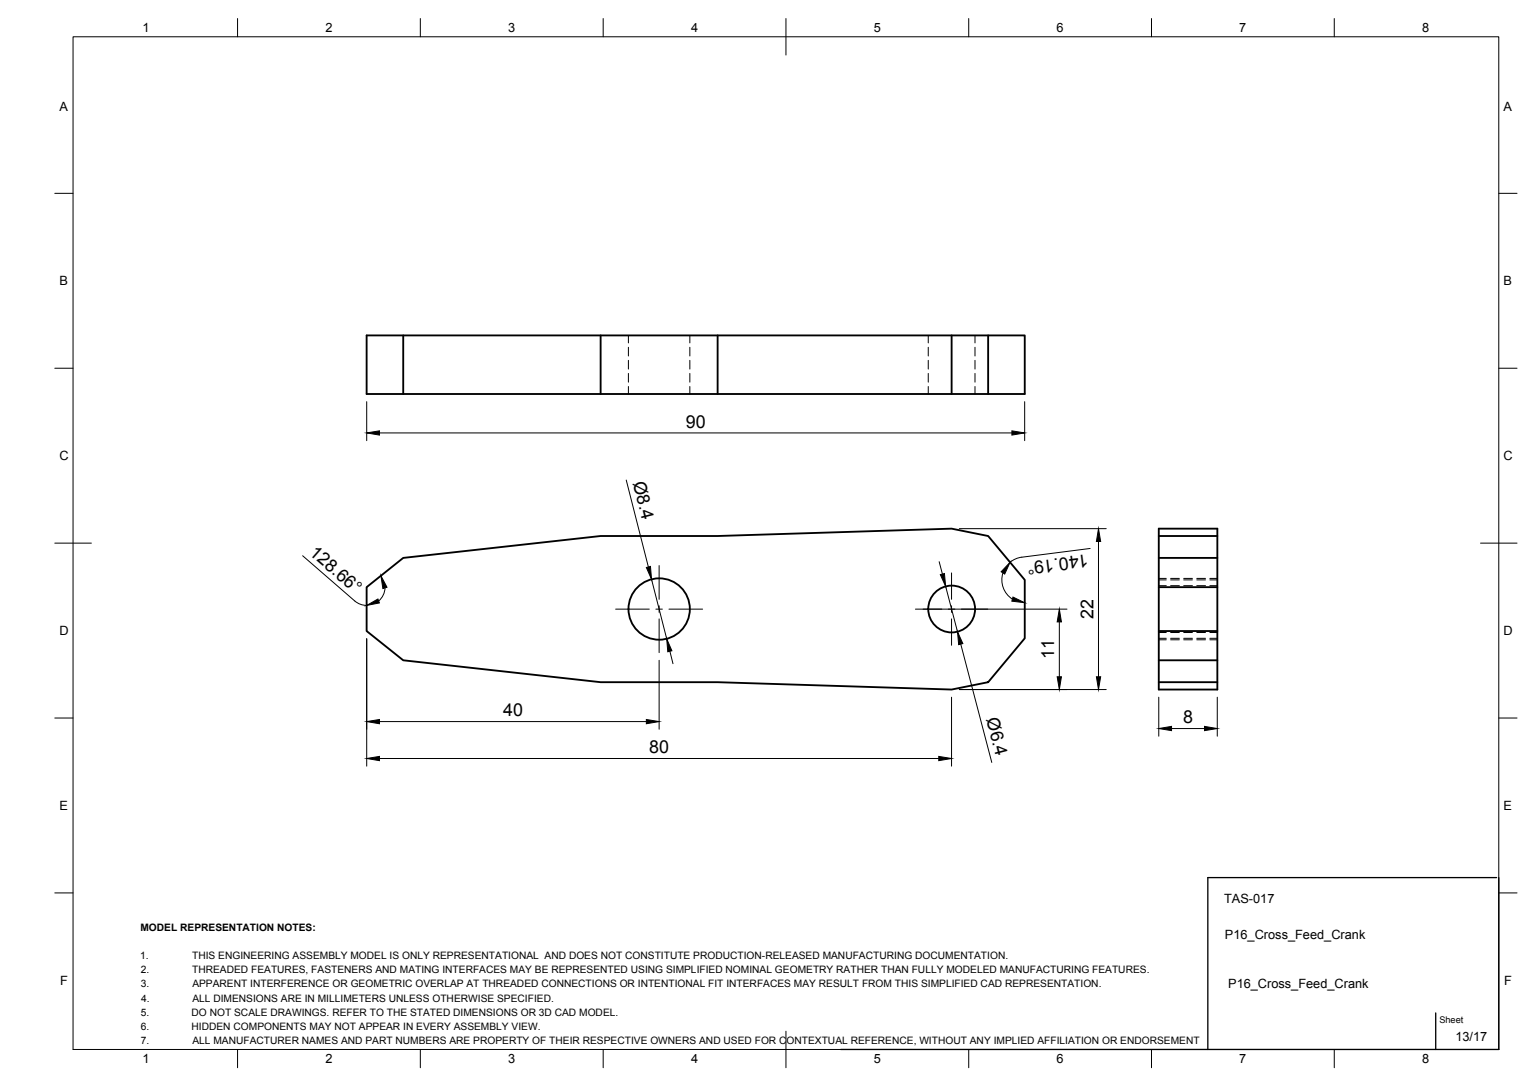
ISO-10303-21;
HEADER;
/* Generated by software containing ST-Developer
 * from STEP Tools, Inc. (www.steptools.com) 
 */

FILE_DESCRIPTION(
/* description */ ('STEP AP203'),
/* implementation_level */ '2;1');

FILE_NAME(
/* name */ 'P16_Cross_Feed_Crank.step',
/* time_stamp */ '2026-11-15T15:04:01-08:00',
/* author */ (''),
/* organization */ (''),
/* preprocessor_version */ 'ST-DEVELOPER v20.2',
/* originating_system */ 'Autodesk Translation Framework v15.17.0.0',
/* authorisation */ '');

FILE_SCHEMA (('AUTOMOTIVE_DESIGN { 1 0 10303 214 3 1 1 }'));
ENDSEC;

DATA;
#10=MECHANICAL_DESIGN_GEOMETRIC_PRESENTATION_REPRESENTATION('',(#299),#16598);
#221=SHAPE_REPRESENTATION_RELATIONSHIP('SRR','None',#16715,#245);
#245=ADVANCED_BREP_SHAPE_REPRESENTATION('',(#269),#16591);
#269=MANIFOLD_SOLID_BREP('Body1',#9804);
#299=STYLED_ITEM('',(#16830),#269);
#415=FACE_BOUND('',#2053,.T.);
#416=FACE_BOUND('',#2054,.T.);
#417=FACE_BOUND('',#2056,.T.);
#418=FACE_BOUND('',#2057,.T.);
#853=PLANE('',#10785);
#854=PLANE('',#10786);
#855=PLANE('',#10787);
#856=PLANE('',#10788);
#857=PLANE('',#10789);
#858=PLANE('',#10790);
#859=PLANE('',#10791);
#860=PLANE('',#10792);
#861=PLANE('',#10793);
#862=PLANE('',#10794);
#863=PLANE('',#10795);
#864=PLANE('',#10796);
#865=PLANE('',#10797);
#866=PLANE('',#10798);
#867=PLANE('',#10799);
#868=PLANE('',#10800);
#1390=FACE_OUTER_BOUND('',#2050,.T.);
#1391=FACE_OUTER_BOUND('',#2051,.T.);
#1392=FACE_OUTER_BOUND('',#2052,.T.);
#1393=FACE_OUTER_BOUND('',#2055,.T.);
#1394=FACE_OUTER_BOUND('',#2058,.T.);
#1395=FACE_OUTER_BOUND('',#2059,.T.);
#1396=FACE_OUTER_BOUND('',#2060,.T.);
#1397=FACE_OUTER_BOUND('',#2061,.T.);
#1398=FACE_OUTER_BOUND('',#2062,.T.);
#1399=FACE_OUTER_BOUND('',#2063,.T.);
#1400=FACE_OUTER_BOUND('',#2064,.T.);
#1401=FACE_OUTER_BOUND('',#2065,.T.);
#1402=FACE_OUTER_BOUND('',#2066,.T.);
#1403=FACE_OUTER_BOUND('',#2067,.T.);
#1404=FACE_OUTER_BOUND('',#2068,.T.);
#1405=FACE_OUTER_BOUND('',#2069,.T.);
#1406=FACE_OUTER_BOUND('',#2070,.T.);
#1407=FACE_OUTER_BOUND('',#2071,.T.);
#2050=EDGE_LOOP('',(#8859,#8860,#8861,#8862));
#2051=EDGE_LOOP('',(#8863,#8864,#8865,#8866));
#2052=EDGE_LOOP('',(#8867,#8868,#8869,#8870,#8871,#8872,#8873,#8874,#8875,
#8876,#8877,#8878,#8879,#8880));
#2053=EDGE_LOOP('',(#8881));
#2054=EDGE_LOOP('',(#8882));
#2055=EDGE_LOOP('',(#8883,#8884,#8885,#8886,#8887,#8888,#8889,#8890,#8891,
#8892,#8893,#8894,#8895,#8896));
#2056=EDGE_LOOP('',(#8897));
#2057=EDGE_LOOP('',(#8898));
#2058=EDGE_LOOP('',(#8899,#8900,#8901,#8902));
#2059=EDGE_LOOP('',(#8903,#8904,#8905,#8906));
#2060=EDGE_LOOP('',(#8907,#8908,#8909,#8910));
#2061=EDGE_LOOP('',(#8911,#8912,#8913,#8914));
#2062=EDGE_LOOP('',(#8915,#8916,#8917,#8918));
#2063=EDGE_LOOP('',(#8919,#8920,#8921,#8922));
#2064=EDGE_LOOP('',(#8923,#8924,#8925,#8926));
#2065=EDGE_LOOP('',(#8927,#8928,#8929,#8930));
#2066=EDGE_LOOP('',(#8931,#8932,#8933,#8934));
#2067=EDGE_LOOP('',(#8935,#8936,#8937,#8938));
#2068=EDGE_LOOP('',(#8939,#8940,#8941,#8942));
#2069=EDGE_LOOP('',(#8943,#8944,#8945,#8946));
#2070=EDGE_LOOP('',(#8947,#8948,#8949,#8950));
#2071=EDGE_LOOP('',(#8951,#8952,#8953,#8954));
#3056=LINE('',#16171,#4104);
#3057=LINE('',#16177,#4105);
#3058=LINE('',#16182,#4106);
#3059=LINE('',#16184,#4107);
#3060=LINE('',#16186,#4108);
#3061=LINE('',#16188,#4109);
#3062=LINE('',#16190,#4110);
#3063=LINE('',#16192,#4111);
#3064=LINE('',#16194,#4112);
#3065=LINE('',#16196,#4113);
#3066=LINE('',#16198,#4114);
#3067=LINE('',#16200,#4115);
#3068=LINE('',#16202,#4116);
#3069=LINE('',#16204,#4117);
#3070=LINE('',#16206,#4118);
#3071=LINE('',#16207,#4119);
#3072=LINE('',#16211,#4120);
#3073=LINE('',#16213,#4121);
#3074=LINE('',#16215,#4122);
#3075=LINE('',#16217,#4123);
#3076=LINE('',#16219,#4124);
#3077=LINE('',#16221,#4125);
#3078=LINE('',#16223,#4126);
#3079=LINE('',#16225,#4127);
#3080=LINE('',#16227,#4128);
#3081=LINE('',#16229,#4129);
#3082=LINE('',#16231,#4130);
#3083=LINE('',#16233,#4131);
#3084=LINE('',#16235,#4132);
#3085=LINE('',#16236,#4133);
#3086=LINE('',#16238,#4134);
#3087=LINE('',#16239,#4135);
#3088=LINE('',#16241,#4136);
#3089=LINE('',#16243,#4137);
#3090=LINE('',#16245,#4138);
#3091=LINE('',#16247,#4139);
#3092=LINE('',#16249,#4140);
#3093=LINE('',#16251,#4141);
#3094=LINE('',#16253,#4142);
#3095=LINE('',#16255,#4143);
#3096=LINE('',#16257,#4144);
#3097=LINE('',#16259,#4145);
#3098=LINE('',#16261,#4146);
#3099=LINE('',#16263,#4147);
#4104=VECTOR('',#13258,3.2);
#4105=VECTOR('',#13265,4.2);
#4106=VECTOR('',#13270,1000.);
#4107=VECTOR('',#13271,1000.);
#4108=VECTOR('',#13272,1000.);
#4109=VECTOR('',#13273,1000.);
#4110=VECTOR('',#13274,1000.);
#4111=VECTOR('',#13275,1000.);
#4112=VECTOR('',#13276,1000.);
#4113=VECTOR('',#13277,1000.);
#4114=VECTOR('',#13278,1000.);
#4115=VECTOR('',#13279,1000.);
#4116=VECTOR('',#13280,1000.);
#4117=VECTOR('',#13281,1000.);
#4118=VECTOR('',#13282,1000.);
#4119=VECTOR('',#13283,1000.);
#4120=VECTOR('',#13286,1000.);
#4121=VECTOR('',#13287,1000.);
#4122=VECTOR('',#13288,1000.);
#4123=VECTOR('',#13289,1000.);
#4124=VECTOR('',#13290,1000.);
#4125=VECTOR('',#13291,1000.);
#4126=VECTOR('',#13292,1000.);
#4127=VECTOR('',#13293,1000.);
#4128=VECTOR('',#13294,1000.);
#4129=VECTOR('',#13295,1000.);
#4130=VECTOR('',#13296,1000.);
#4131=VECTOR('',#13297,1000.);
#4132=VECTOR('',#13298,1000.);
#4133=VECTOR('',#13299,1000.);
#4134=VECTOR('',#13302,1000.);
#4135=VECTOR('',#13303,1000.);
#4136=VECTOR('',#13306,1000.);
#4137=VECTOR('',#13309,1000.);
#4138=VECTOR('',#13312,1000.);
#4139=VECTOR('',#13315,1000.);
#4140=VECTOR('',#13318,1000.);
#4141=VECTOR('',#13321,1000.);
#4142=VECTOR('',#13324,1000.);
#4143=VECTOR('',#13327,1000.);
#4144=VECTOR('',#13330,1000.);
#4145=VECTOR('',#13333,1000.);
#4146=VECTOR('',#13336,1000.);
#4147=VECTOR('',#13339,1000.);
#4428=CIRCLE('',#10780,3.2);
#4429=CIRCLE('',#10781,3.2);
#4430=CIRCLE('',#10783,4.2);
#4431=CIRCLE('',#10784,4.2);
#5208=VERTEX_POINT('',#16168);
#5209=VERTEX_POINT('',#16170);
#5210=VERTEX_POINT('',#16174);
#5211=VERTEX_POINT('',#16176);
#5212=VERTEX_POINT('',#16180);
#5213=VERTEX_POINT('',#16181);
#5214=VERTEX_POINT('',#16183);
#5215=VERTEX_POINT('',#16185);
#5216=VERTEX_POINT('',#16187);
#5217=VERTEX_POINT('',#16189);
#5218=VERTEX_POINT('',#16191);
#5219=VERTEX_POINT('',#16193);
#5220=VERTEX_POINT('',#16195);
#5221=VERTEX_POINT('',#16197);
#5222=VERTEX_POINT('',#16199);
#5223=VERTEX_POINT('',#16201);
#5224=VERTEX_POINT('',#16203);
#5225=VERTEX_POINT('',#16205);
#5226=VERTEX_POINT('',#16209);
#5227=VERTEX_POINT('',#16210);
#5228=VERTEX_POINT('',#16212);
#5229=VERTEX_POINT('',#16214);
#5230=VERTEX_POINT('',#16216);
#5231=VERTEX_POINT('',#16218);
#5232=VERTEX_POINT('',#16220);
#5233=VERTEX_POINT('',#16222);
#5234=VERTEX_POINT('',#16224);
#5235=VERTEX_POINT('',#16226);
#5236=VERTEX_POINT('',#16228);
#5237=VERTEX_POINT('',#16230);
#5238=VERTEX_POINT('',#16232);
#5239=VERTEX_POINT('',#16234);
#6442=EDGE_CURVE('',#5208,#5208,#4428,.T.);
#6443=EDGE_CURVE('',#5208,#5209,#3056,.T.);
#6444=EDGE_CURVE('',#5209,#5209,#4429,.T.);
#6445=EDGE_CURVE('',#5210,#5210,#4430,.T.);
#6446=EDGE_CURVE('',#5210,#5211,#3057,.T.);
#6447=EDGE_CURVE('',#5211,#5211,#4431,.T.);
#6448=EDGE_CURVE('',#5212,#5213,#3058,.T.);
#6449=EDGE_CURVE('',#5213,#5214,#3059,.T.);
#6450=EDGE_CURVE('',#5214,#5215,#3060,.T.);
#6451=EDGE_CURVE('',#5215,#5216,#3061,.T.);
#6452=EDGE_CURVE('',#5216,#5217,#3062,.T.);
#6453=EDGE_CURVE('',#5217,#5218,#3063,.T.);
#6454=EDGE_CURVE('',#5218,#5219,#3064,.T.);
#6455=EDGE_CURVE('',#5219,#5220,#3065,.T.);
#6456=EDGE_CURVE('',#5220,#5221,#3066,.T.);
#6457=EDGE_CURVE('',#5221,#5222,#3067,.T.);
#6458=EDGE_CURVE('',#5222,#5223,#3068,.T.);
#6459=EDGE_CURVE('',#5223,#5224,#3069,.T.);
#6460=EDGE_CURVE('',#5224,#5225,#3070,.T.);
#6461=EDGE_CURVE('',#5225,#5212,#3071,.T.);
#6462=EDGE_CURVE('',#5226,#5227,#3072,.T.);
#6463=EDGE_CURVE('',#5228,#5226,#3073,.T.);
#6464=EDGE_CURVE('',#5229,#5228,#3074,.T.);
#6465=EDGE_CURVE('',#5230,#5229,#3075,.T.);
#6466=EDGE_CURVE('',#5231,#5230,#3076,.T.);
#6467=EDGE_CURVE('',#5232,#5231,#3077,.T.);
#6468=EDGE_CURVE('',#5233,#5232,#3078,.T.);
#6469=EDGE_CURVE('',#5234,#5233,#3079,.T.);
#6470=EDGE_CURVE('',#5235,#5234,#3080,.T.);
#6471=EDGE_CURVE('',#5236,#5235,#3081,.T.);
#6472=EDGE_CURVE('',#5237,#5236,#3082,.T.);
#6473=EDGE_CURVE('',#5238,#5237,#3083,.T.);
#6474=EDGE_CURVE('',#5239,#5238,#3084,.T.);
#6475=EDGE_CURVE('',#5227,#5239,#3085,.T.);
#6476=EDGE_CURVE('',#5213,#5227,#3086,.T.);
#6477=EDGE_CURVE('',#5212,#5226,#3087,.T.);
#6478=EDGE_CURVE('',#5214,#5239,#3088,.T.);
#6479=EDGE_CURVE('',#5215,#5238,#3089,.T.);
#6480=EDGE_CURVE('',#5216,#5237,#3090,.T.);
#6481=EDGE_CURVE('',#5217,#5236,#3091,.T.);
#6482=EDGE_CURVE('',#5218,#5235,#3092,.T.);
#6483=EDGE_CURVE('',#5219,#5234,#3093,.T.);
#6484=EDGE_CURVE('',#5220,#5233,#3094,.T.);
#6485=EDGE_CURVE('',#5221,#5232,#3095,.T.);
#6486=EDGE_CURVE('',#5222,#5231,#3096,.T.);
#6487=EDGE_CURVE('',#5223,#5230,#3097,.T.);
#6488=EDGE_CURVE('',#5224,#5229,#3098,.T.);
#6489=EDGE_CURVE('',#5225,#5228,#3099,.T.);
#8859=ORIENTED_EDGE('',*,*,#6442,.T.);
#8860=ORIENTED_EDGE('',*,*,#6443,.T.);
#8861=ORIENTED_EDGE('',*,*,#6444,.F.);
#8862=ORIENTED_EDGE('',*,*,#6443,.F.);
#8863=ORIENTED_EDGE('',*,*,#6445,.T.);
#8864=ORIENTED_EDGE('',*,*,#6446,.T.);
#8865=ORIENTED_EDGE('',*,*,#6447,.F.);
#8866=ORIENTED_EDGE('',*,*,#6446,.F.);
#8867=ORIENTED_EDGE('',*,*,#6448,.T.);
#8868=ORIENTED_EDGE('',*,*,#6449,.T.);
#8869=ORIENTED_EDGE('',*,*,#6450,.T.);
#8870=ORIENTED_EDGE('',*,*,#6451,.T.);
#8871=ORIENTED_EDGE('',*,*,#6452,.T.);
#8872=ORIENTED_EDGE('',*,*,#6453,.T.);
#8873=ORIENTED_EDGE('',*,*,#6454,.T.);
#8874=ORIENTED_EDGE('',*,*,#6455,.T.);
#8875=ORIENTED_EDGE('',*,*,#6456,.T.);
#8876=ORIENTED_EDGE('',*,*,#6457,.T.);
#8877=ORIENTED_EDGE('',*,*,#6458,.T.);
#8878=ORIENTED_EDGE('',*,*,#6459,.T.);
#8879=ORIENTED_EDGE('',*,*,#6460,.T.);
#8880=ORIENTED_EDGE('',*,*,#6461,.T.);
#8881=ORIENTED_EDGE('',*,*,#6442,.F.);
#8882=ORIENTED_EDGE('',*,*,#6445,.F.);
#8883=ORIENTED_EDGE('',*,*,#6462,.F.);
#8884=ORIENTED_EDGE('',*,*,#6463,.F.);
#8885=ORIENTED_EDGE('',*,*,#6464,.F.);
#8886=ORIENTED_EDGE('',*,*,#6465,.F.);
#8887=ORIENTED_EDGE('',*,*,#6466,.F.);
#8888=ORIENTED_EDGE('',*,*,#6467,.F.);
#8889=ORIENTED_EDGE('',*,*,#6468,.F.);
#8890=ORIENTED_EDGE('',*,*,#6469,.F.);
#8891=ORIENTED_EDGE('',*,*,#6470,.F.);
#8892=ORIENTED_EDGE('',*,*,#6471,.F.);
#8893=ORIENTED_EDGE('',*,*,#6472,.F.);
#8894=ORIENTED_EDGE('',*,*,#6473,.F.);
#8895=ORIENTED_EDGE('',*,*,#6474,.F.);
#8896=ORIENTED_EDGE('',*,*,#6475,.F.);
#8897=ORIENTED_EDGE('',*,*,#6447,.T.);
#8898=ORIENTED_EDGE('',*,*,#6444,.T.);
#8899=ORIENTED_EDGE('',*,*,#6462,.T.);
#8900=ORIENTED_EDGE('',*,*,#6476,.F.);
#8901=ORIENTED_EDGE('',*,*,#6448,.F.);
#8902=ORIENTED_EDGE('',*,*,#6477,.T.);
#8903=ORIENTED_EDGE('',*,*,#6475,.T.);
#8904=ORIENTED_EDGE('',*,*,#6478,.F.);
#8905=ORIENTED_EDGE('',*,*,#6449,.F.);
#8906=ORIENTED_EDGE('',*,*,#6476,.T.);
#8907=ORIENTED_EDGE('',*,*,#6474,.T.);
#8908=ORIENTED_EDGE('',*,*,#6479,.F.);
#8909=ORIENTED_EDGE('',*,*,#6450,.F.);
#8910=ORIENTED_EDGE('',*,*,#6478,.T.);
#8911=ORIENTED_EDGE('',*,*,#6473,.T.);
#8912=ORIENTED_EDGE('',*,*,#6480,.F.);
#8913=ORIENTED_EDGE('',*,*,#6451,.F.);
#8914=ORIENTED_EDGE('',*,*,#6479,.T.);
#8915=ORIENTED_EDGE('',*,*,#6472,.T.);
#8916=ORIENTED_EDGE('',*,*,#6481,.F.);
#8917=ORIENTED_EDGE('',*,*,#6452,.F.);
#8918=ORIENTED_EDGE('',*,*,#6480,.T.);
#8919=ORIENTED_EDGE('',*,*,#6471,.T.);
#8920=ORIENTED_EDGE('',*,*,#6482,.F.);
#8921=ORIENTED_EDGE('',*,*,#6453,.F.);
#8922=ORIENTED_EDGE('',*,*,#6481,.T.);
#8923=ORIENTED_EDGE('',*,*,#6470,.T.);
#8924=ORIENTED_EDGE('',*,*,#6483,.F.);
#8925=ORIENTED_EDGE('',*,*,#6454,.F.);
#8926=ORIENTED_EDGE('',*,*,#6482,.T.);
#8927=ORIENTED_EDGE('',*,*,#6469,.T.);
#8928=ORIENTED_EDGE('',*,*,#6484,.F.);
#8929=ORIENTED_EDGE('',*,*,#6455,.F.);
#8930=ORIENTED_EDGE('',*,*,#6483,.T.);
#8931=ORIENTED_EDGE('',*,*,#6468,.T.);
#8932=ORIENTED_EDGE('',*,*,#6485,.F.);
#8933=ORIENTED_EDGE('',*,*,#6456,.F.);
#8934=ORIENTED_EDGE('',*,*,#6484,.T.);
#8935=ORIENTED_EDGE('',*,*,#6467,.T.);
#8936=ORIENTED_EDGE('',*,*,#6486,.F.);
#8937=ORIENTED_EDGE('',*,*,#6457,.F.);
#8938=ORIENTED_EDGE('',*,*,#6485,.T.);
#8939=ORIENTED_EDGE('',*,*,#6466,.T.);
#8940=ORIENTED_EDGE('',*,*,#6487,.F.);
#8941=ORIENTED_EDGE('',*,*,#6458,.F.);
#8942=ORIENTED_EDGE('',*,*,#6486,.T.);
#8943=ORIENTED_EDGE('',*,*,#6465,.T.);
#8944=ORIENTED_EDGE('',*,*,#6488,.F.);
#8945=ORIENTED_EDGE('',*,*,#6459,.F.);
#8946=ORIENTED_EDGE('',*,*,#6487,.T.);
#8947=ORIENTED_EDGE('',*,*,#6464,.T.);
#8948=ORIENTED_EDGE('',*,*,#6489,.F.);
#8949=ORIENTED_EDGE('',*,*,#6460,.F.);
#8950=ORIENTED_EDGE('',*,*,#6488,.T.);
#8951=ORIENTED_EDGE('',*,*,#6463,.T.);
#8952=ORIENTED_EDGE('',*,*,#6477,.F.);
#8953=ORIENTED_EDGE('',*,*,#6461,.F.);
#8954=ORIENTED_EDGE('',*,*,#6489,.T.);
#9224=CYLINDRICAL_SURFACE('',#10779,3.2);
#9225=CYLINDRICAL_SURFACE('',#10782,4.2);
#9715=ADVANCED_FACE('',(#1390),#9224,.F.);
#9716=ADVANCED_FACE('',(#1391),#9225,.F.);
#9717=ADVANCED_FACE('',(#1392,#415,#416),#853,.T.);
#9718=ADVANCED_FACE('',(#1393,#417,#418),#854,.F.);
#9719=ADVANCED_FACE('',(#1394),#855,.F.);
#9720=ADVANCED_FACE('',(#1395),#856,.F.);
#9721=ADVANCED_FACE('',(#1396),#857,.F.);
#9722=ADVANCED_FACE('',(#1397),#858,.F.);
#9723=ADVANCED_FACE('',(#1398),#859,.F.);
#9724=ADVANCED_FACE('',(#1399),#860,.F.);
#9725=ADVANCED_FACE('',(#1400),#861,.F.);
#9726=ADVANCED_FACE('',(#1401),#862,.F.);
#9727=ADVANCED_FACE('',(#1402),#863,.F.);
#9728=ADVANCED_FACE('',(#1403),#864,.F.);
#9729=ADVANCED_FACE('',(#1404),#865,.F.);
#9730=ADVANCED_FACE('',(#1405),#866,.F.);
#9731=ADVANCED_FACE('',(#1406),#867,.F.);
#9732=ADVANCED_FACE('',(#1407),#868,.F.);
#9804=CLOSED_SHELL('',(#9715,#9716,#9717,#9718,#9719,#9720,#9721,#9722,
#9723,#9724,#9725,#9726,#9727,#9728,#9729,#9730,#9731,#9732));
#10778=AXIS2_PLACEMENT_3D('',#16166,#13252,#13253);
#10779=AXIS2_PLACEMENT_3D('',#16167,#13254,#13255);
#10780=AXIS2_PLACEMENT_3D('',#16169,#13256,#13257);
#10781=AXIS2_PLACEMENT_3D('',#16172,#13259,#13260);
#10782=AXIS2_PLACEMENT_3D('',#16173,#13261,#13262);
#10783=AXIS2_PLACEMENT_3D('',#16175,#13263,#13264);
#10784=AXIS2_PLACEMENT_3D('',#16178,#13266,#13267);
#10785=AXIS2_PLACEMENT_3D('',#16179,#13268,#13269);
#10786=AXIS2_PLACEMENT_3D('',#16208,#13284,#13285);
#10787=AXIS2_PLACEMENT_3D('',#16237,#13300,#13301);
#10788=AXIS2_PLACEMENT_3D('',#16240,#13304,#13305);
#10789=AXIS2_PLACEMENT_3D('',#16242,#13307,#13308);
#10790=AXIS2_PLACEMENT_3D('',#16244,#13310,#13311);
#10791=AXIS2_PLACEMENT_3D('',#16246,#13313,#13314);
#10792=AXIS2_PLACEMENT_3D('',#16248,#13316,#13317);
#10793=AXIS2_PLACEMENT_3D('',#16250,#13319,#13320);
#10794=AXIS2_PLACEMENT_3D('',#16252,#13322,#13323);
#10795=AXIS2_PLACEMENT_3D('',#16254,#13325,#13326);
#10796=AXIS2_PLACEMENT_3D('',#16256,#13328,#13329);
#10797=AXIS2_PLACEMENT_3D('',#16258,#13331,#13332);
#10798=AXIS2_PLACEMENT_3D('',#16260,#13334,#13335);
#10799=AXIS2_PLACEMENT_3D('',#16262,#13337,#13338);
#10800=AXIS2_PLACEMENT_3D('',#16264,#13340,#13341);
#13252=DIRECTION('axis',(0.,0.,1.));
#13253=DIRECTION('refdir',(1.,0.,0.));
#13254=DIRECTION('center_axis',(0.,0.,-1.));
#13255=DIRECTION('ref_axis',(-1.,0.,0.));
#13256=DIRECTION('center_axis',(0.,0.,1.));
#13257=DIRECTION('ref_axis',(1.,0.,0.));
#13258=DIRECTION('',(0.,0.,-1.));
#13259=DIRECTION('center_axis',(0.,0.,1.));
#13260=DIRECTION('ref_axis',(1.,0.,0.));
#13261=DIRECTION('center_axis',(0.,0.,-1.));
#13262=DIRECTION('ref_axis',(-1.,0.,0.));
#13263=DIRECTION('center_axis',(0.,0.,1.));
#13264=DIRECTION('ref_axis',(1.,0.,0.));
#13265=DIRECTION('',(0.,0.,-1.));
#13266=DIRECTION('center_axis',(0.,0.,1.));
#13267=DIRECTION('ref_axis',(1.,0.,0.));
#13268=DIRECTION('center_axis',(0.,0.,1.));
#13269=DIRECTION('ref_axis',(1.,0.,0.));
#13270=DIRECTION('',(0.,-1.,0.));
#13271=DIRECTION('',(0.64018439966448,-0.768221279597376,0.));
#13272=DIRECTION('',(0.98058067569092,-0.196116135138184,0.));
#13273=DIRECTION('',(0.999512076087079,0.0312347523777212,0.));
#13274=DIRECTION('',(1.,0.,0.));
#13275=DIRECTION('',(0.993883734673619,0.110431526074847,0.));
#13276=DIRECTION('',(0.78086880944303,0.624695047554424,0.));
#13277=DIRECTION('',(0.,1.,0.));
#13278=DIRECTION('',(-0.78086880944303,0.624695047554424,0.));
#13279=DIRECTION('',(-0.993883734673619,0.110431526074847,0.));
#13280=DIRECTION('',(-1.,0.,0.));
#13281=DIRECTION('',(-0.999512076087079,0.0312347523777212,0.));
#13282=DIRECTION('',(-0.98058067569092,-0.196116135138184,0.));
#13283=DIRECTION('',(-0.64018439966448,-0.768221279597376,0.));
#13284=DIRECTION('center_axis',(0.,0.,1.));
#13285=DIRECTION('ref_axis',(1.,0.,0.));
#13286=DIRECTION('',(0.,-1.,0.));
#13287=DIRECTION('',(-0.64018439966448,-0.768221279597376,0.));
#13288=DIRECTION('',(-0.98058067569092,-0.196116135138184,0.));
#13289=DIRECTION('',(-0.999512076087079,0.0312347523777212,0.));
#13290=DIRECTION('',(-1.,0.,0.));
#13291=DIRECTION('',(-0.993883734673619,0.110431526074847,0.));
#13292=DIRECTION('',(-0.78086880944303,0.624695047554424,0.));
#13293=DIRECTION('',(0.,1.,0.));
#13294=DIRECTION('',(0.78086880944303,0.624695047554424,0.));
#13295=DIRECTION('',(0.993883734673619,0.110431526074847,0.));
#13296=DIRECTION('',(1.,0.,0.));
#13297=DIRECTION('',(0.999512076087079,0.0312347523777212,0.));
#13298=DIRECTION('',(0.98058067569092,-0.196116135138184,0.));
#13299=DIRECTION('',(0.64018439966448,-0.768221279597376,0.));
#13300=DIRECTION('center_axis',(1.,0.,0.));
#13301=DIRECTION('ref_axis',(0.,0.,-1.));
#13302=DIRECTION('',(0.,0.,-1.));
#13303=DIRECTION('',(0.,0.,-1.));
#13304=DIRECTION('center_axis',(0.768221279597376,0.64018439966448,0.));
#13305=DIRECTION('ref_axis',(-0.64018439966448,0.768221279597376,0.));
#13306=DIRECTION('',(0.,0.,-1.));
#13307=DIRECTION('center_axis',(0.196116135138184,0.98058067569092,0.));
#13308=DIRECTION('ref_axis',(-0.98058067569092,0.196116135138184,0.));
#13309=DIRECTION('',(0.,0.,-1.));
#13310=DIRECTION('center_axis',(-0.0312347523777212,0.999512076087079,0.));
#13311=DIRECTION('ref_axis',(-0.999512076087079,-0.0312347523777212,0.));
#13312=DIRECTION('',(0.,0.,-1.));
#13313=DIRECTION('center_axis',(0.,1.,0.));
#13314=DIRECTION('ref_axis',(0.,0.,1.));
#13315=DIRECTION('',(0.,0.,-1.));
#13316=DIRECTION('center_axis',(-0.110431526074847,0.993883734673619,0.));
#13317=DIRECTION('ref_axis',(-0.993883734673619,-0.110431526074847,0.));
#13318=DIRECTION('',(0.,0.,-1.));
#13319=DIRECTION('center_axis',(-0.624695047554425,0.78086880944303,0.));
#13320=DIRECTION('ref_axis',(-0.78086880944303,-0.624695047554424,0.));
#13321=DIRECTION('',(0.,0.,-1.));
#13322=DIRECTION('center_axis',(-1.,0.,0.));
#13323=DIRECTION('ref_axis',(0.,0.,1.));
#13324=DIRECTION('',(0.,0.,-1.));
#13325=DIRECTION('center_axis',(-0.624695047554425,-0.78086880944303,0.));
#13326=DIRECTION('ref_axis',(0.78086880944303,-0.624695047554424,0.));
#13327=DIRECTION('',(0.,0.,-1.));
#13328=DIRECTION('center_axis',(-0.110431526074847,-0.993883734673619,0.));
#13329=DIRECTION('ref_axis',(0.993883734673619,-0.110431526074847,0.));
#13330=DIRECTION('',(0.,0.,-1.));
#13331=DIRECTION('center_axis',(0.,-1.,0.));
#13332=DIRECTION('ref_axis',(0.,0.,-1.));
#13333=DIRECTION('',(0.,0.,-1.));
#13334=DIRECTION('center_axis',(-0.0312347523777212,-0.999512076087079,
0.));
#13335=DIRECTION('ref_axis',(0.999512076087079,-0.0312347523777212,0.));
#13336=DIRECTION('',(0.,0.,-1.));
#13337=DIRECTION('center_axis',(0.196116135138184,-0.98058067569092,0.));
#13338=DIRECTION('ref_axis',(0.98058067569092,0.196116135138184,0.));
#13339=DIRECTION('',(0.,0.,-1.));
#13340=DIRECTION('center_axis',(0.768221279597376,-0.64018439966448,0.));
#13341=DIRECTION('ref_axis',(0.64018439966448,0.768221279597376,0.));
#16166=CARTESIAN_POINT('',(0.,0.,0.));
#16167=CARTESIAN_POINT('Origin',(-40.,0.,8.));
#16168=CARTESIAN_POINT('',(-36.8,-3.91886975727153E-16,8.));
#16169=CARTESIAN_POINT('Origin',(-40.,0.,8.));
#16170=CARTESIAN_POINT('',(-36.8,-3.91886975727153E-16,0.));
#16171=CARTESIAN_POINT('',(-36.8,-3.91886975727153E-16,8.));
#16172=CARTESIAN_POINT('Origin',(-40.,0.,0.));
#16173=CARTESIAN_POINT('Origin',(0.,0.,8.));
#16174=CARTESIAN_POINT('',(4.2,-5.14351655641888E-16,8.));
#16175=CARTESIAN_POINT('Origin',(0.,0.,8.));
#16176=CARTESIAN_POINT('',(4.2,-5.14351655641888E-16,0.));
#16177=CARTESIAN_POINT('',(4.2,-5.14351655641888E-16,8.));
#16178=CARTESIAN_POINT('Origin',(0.,0.,0.));
#16179=CARTESIAN_POINT('Origin',(0.,0.,8.));
#16180=CARTESIAN_POINT('',(-50.,4.,8.));
#16181=CARTESIAN_POINT('',(-50.,-4.,8.));
#16182=CARTESIAN_POINT('',(-50.,4.,8.));
#16183=CARTESIAN_POINT('',(-45.,-10.,8.));
#16184=CARTESIAN_POINT('',(-50.,-4.,8.));
#16185=CARTESIAN_POINT('',(-40.,-11.,8.));
#16186=CARTESIAN_POINT('',(-45.,-10.,8.));
#16187=CARTESIAN_POINT('',(-8.,-10.,8.));
#16188=CARTESIAN_POINT('',(-40.,-11.,8.));
#16189=CARTESIAN_POINT('',(8.,-10.,8.));
#16190=CARTESIAN_POINT('',(-8.,-10.,8.));
#16191=CARTESIAN_POINT('',(35.,-7.,8.));
#16192=CARTESIAN_POINT('',(8.,-10.,8.));
#16193=CARTESIAN_POINT('',(40.,-3.,8.));
#16194=CARTESIAN_POINT('',(35.,-7.,8.));
#16195=CARTESIAN_POINT('',(40.,3.,8.));
#16196=CARTESIAN_POINT('',(40.,-3.,8.));
#16197=CARTESIAN_POINT('',(35.,7.,8.));
#16198=CARTESIAN_POINT('',(40.,3.,8.));
#16199=CARTESIAN_POINT('',(8.,10.,8.));
#16200=CARTESIAN_POINT('',(35.,7.,8.));
#16201=CARTESIAN_POINT('',(-8.,10.,8.));
#16202=CARTESIAN_POINT('',(8.,10.,8.));
#16203=CARTESIAN_POINT('',(-40.,11.,8.));
#16204=CARTESIAN_POINT('',(-8.,10.,8.));
#16205=CARTESIAN_POINT('',(-45.,10.,8.));
#16206=CARTESIAN_POINT('',(-40.,11.,8.));
#16207=CARTESIAN_POINT('',(-45.,10.,8.));
#16208=CARTESIAN_POINT('Origin',(0.,0.,0.));
#16209=CARTESIAN_POINT('',(-50.,4.,0.));
#16210=CARTESIAN_POINT('',(-50.,-4.,0.));
#16211=CARTESIAN_POINT('',(-50.,4.,0.));
#16212=CARTESIAN_POINT('',(-45.,10.,0.));
#16213=CARTESIAN_POINT('',(-45.,10.,0.));
#16214=CARTESIAN_POINT('',(-40.,11.,0.));
#16215=CARTESIAN_POINT('',(-40.,11.,0.));
#16216=CARTESIAN_POINT('',(-8.,10.,0.));
#16217=CARTESIAN_POINT('',(-8.,10.,0.));
#16218=CARTESIAN_POINT('',(8.,10.,0.));
#16219=CARTESIAN_POINT('',(8.,10.,0.));
#16220=CARTESIAN_POINT('',(35.,7.,0.));
#16221=CARTESIAN_POINT('',(35.,7.,0.));
#16222=CARTESIAN_POINT('',(40.,3.,0.));
#16223=CARTESIAN_POINT('',(40.,3.,0.));
#16224=CARTESIAN_POINT('',(40.,-3.,0.));
#16225=CARTESIAN_POINT('',(40.,-3.,0.));
#16226=CARTESIAN_POINT('',(35.,-7.,0.));
#16227=CARTESIAN_POINT('',(35.,-7.,0.));
#16228=CARTESIAN_POINT('',(8.,-10.,0.));
#16229=CARTESIAN_POINT('',(8.,-10.,0.));
#16230=CARTESIAN_POINT('',(-8.,-10.,0.));
#16231=CARTESIAN_POINT('',(-8.,-10.,0.));
#16232=CARTESIAN_POINT('',(-40.,-11.,0.));
#16233=CARTESIAN_POINT('',(-40.,-11.,0.));
#16234=CARTESIAN_POINT('',(-45.,-10.,0.));
#16235=CARTESIAN_POINT('',(-45.,-10.,0.));
#16236=CARTESIAN_POINT('',(-50.,-4.,0.));
#16237=CARTESIAN_POINT('Origin',(-50.,4.,8.));
#16238=CARTESIAN_POINT('',(-50.,-4.,8.));
#16239=CARTESIAN_POINT('',(-50.,4.,8.));
#16240=CARTESIAN_POINT('Origin',(-50.,-4.,8.));
#16241=CARTESIAN_POINT('',(-45.,-10.,8.));
#16242=CARTESIAN_POINT('Origin',(-45.,-10.,8.));
#16243=CARTESIAN_POINT('',(-40.,-11.,8.));
#16244=CARTESIAN_POINT('Origin',(-40.,-11.,8.));
#16245=CARTESIAN_POINT('',(-8.,-10.,8.));
#16246=CARTESIAN_POINT('Origin',(-8.,-10.,8.));
#16247=CARTESIAN_POINT('',(8.,-10.,8.));
#16248=CARTESIAN_POINT('Origin',(8.,-10.,8.));
#16249=CARTESIAN_POINT('',(35.,-7.,8.));
#16250=CARTESIAN_POINT('Origin',(35.,-7.,8.));
#16251=CARTESIAN_POINT('',(40.,-3.,8.));
#16252=CARTESIAN_POINT('Origin',(40.,-3.,8.));
#16253=CARTESIAN_POINT('',(40.,3.,8.));
#16254=CARTESIAN_POINT('Origin',(40.,3.,8.));
#16255=CARTESIAN_POINT('',(35.,7.,8.));
#16256=CARTESIAN_POINT('Origin',(35.,7.,8.));
#16257=CARTESIAN_POINT('',(8.,10.,8.));
#16258=CARTESIAN_POINT('Origin',(8.,10.,8.));
#16259=CARTESIAN_POINT('',(-8.,10.,8.));
#16260=CARTESIAN_POINT('Origin',(-8.,10.,8.));
#16261=CARTESIAN_POINT('',(-40.,11.,8.));
#16262=CARTESIAN_POINT('Origin',(-40.,11.,8.));
#16263=CARTESIAN_POINT('',(-45.,10.,8.));
#16264=CARTESIAN_POINT('Origin',(-45.,10.,8.));
#16565=UNCERTAINTY_MEASURE_WITH_UNIT(LENGTH_MEASURE(0.01),#16599,
'DISTANCE_ACCURACY_VALUE',
'Maximum model space distance between geometric entities at asserted c
onnectivities');
#16572=UNCERTAINTY_MEASURE_WITH_UNIT(LENGTH_MEASURE(0.01),#16599,
'DISTANCE_ACCURACY_VALUE',
'Maximum model space distance between geometric entities at asserted c
onnectivities');
#16591=(
GEOMETRIC_REPRESENTATION_CONTEXT(3)
GLOBAL_UNCERTAINTY_ASSIGNED_CONTEXT((#16565))
GLOBAL_UNIT_ASSIGNED_CONTEXT((#16599,#16601,#16602))
REPRESENTATION_CONTEXT('','3D')
);
#16598=(
GEOMETRIC_REPRESENTATION_CONTEXT(3)
GLOBAL_UNCERTAINTY_ASSIGNED_CONTEXT((#16572))
GLOBAL_UNIT_ASSIGNED_CONTEXT((#16599,#16601,#16602))
REPRESENTATION_CONTEXT('','3D')
);
#16599=(
LENGTH_UNIT()
NAMED_UNIT(*)
SI_UNIT(.MILLI.,.METRE.)
);
#16601=(
NAMED_UNIT(*)
PLANE_ANGLE_UNIT()
SI_UNIT($,.RADIAN.)
);
#16602=(
NAMED_UNIT(*)
SI_UNIT($,.STERADIAN.)
SOLID_ANGLE_UNIT()
);
#16621=SHAPE_DEFINITION_REPRESENTATION(#16646,#16715);
#16646=PRODUCT_DEFINITION_SHAPE('',$,#16741);
#16715=SHAPE_REPRESENTATION('',(#10778),#16591);
#16722=PRODUCT_DEFINITION_CONTEXT('part definition',#16799,'design');
#16741=PRODUCT_DEFINITION('P16_Cross_Feed_Crank','P16_Cross_Feed_Crank',
#16766,#16722);
#16766=PRODUCT_DEFINITION_FORMATION('',$,#16819);
#16799=APPLICATION_CONTEXT(
'Core Data for Automotive Mechanical Design Process');
#16800=PRODUCT_CONTEXT('part definition',#16799,'mechanical');
#16819=PRODUCT('P16_Cross_Feed_Crank','P16_Cross_Feed_Crank',$,(#16800));
#16830=PRESENTATION_STYLE_ASSIGNMENT((#16839));
#16839=SURFACE_STYLE_USAGE(.BOTH.,#16848);
#16848=SURFACE_SIDE_STYLE('',(#16857));
#16857=SURFACE_STYLE_FILL_AREA(#16866);
#16866=FILL_AREA_STYLE('Dark Blue',(#16875));
#16875=FILL_AREA_STYLE_COLOUR('Dark Blue',#16884);
#16884=COLOUR_RGB('Dark Blue',0.,0.125490196078431,0.376470588235294);
ENDSEC;
END-ISO-10303-21;
